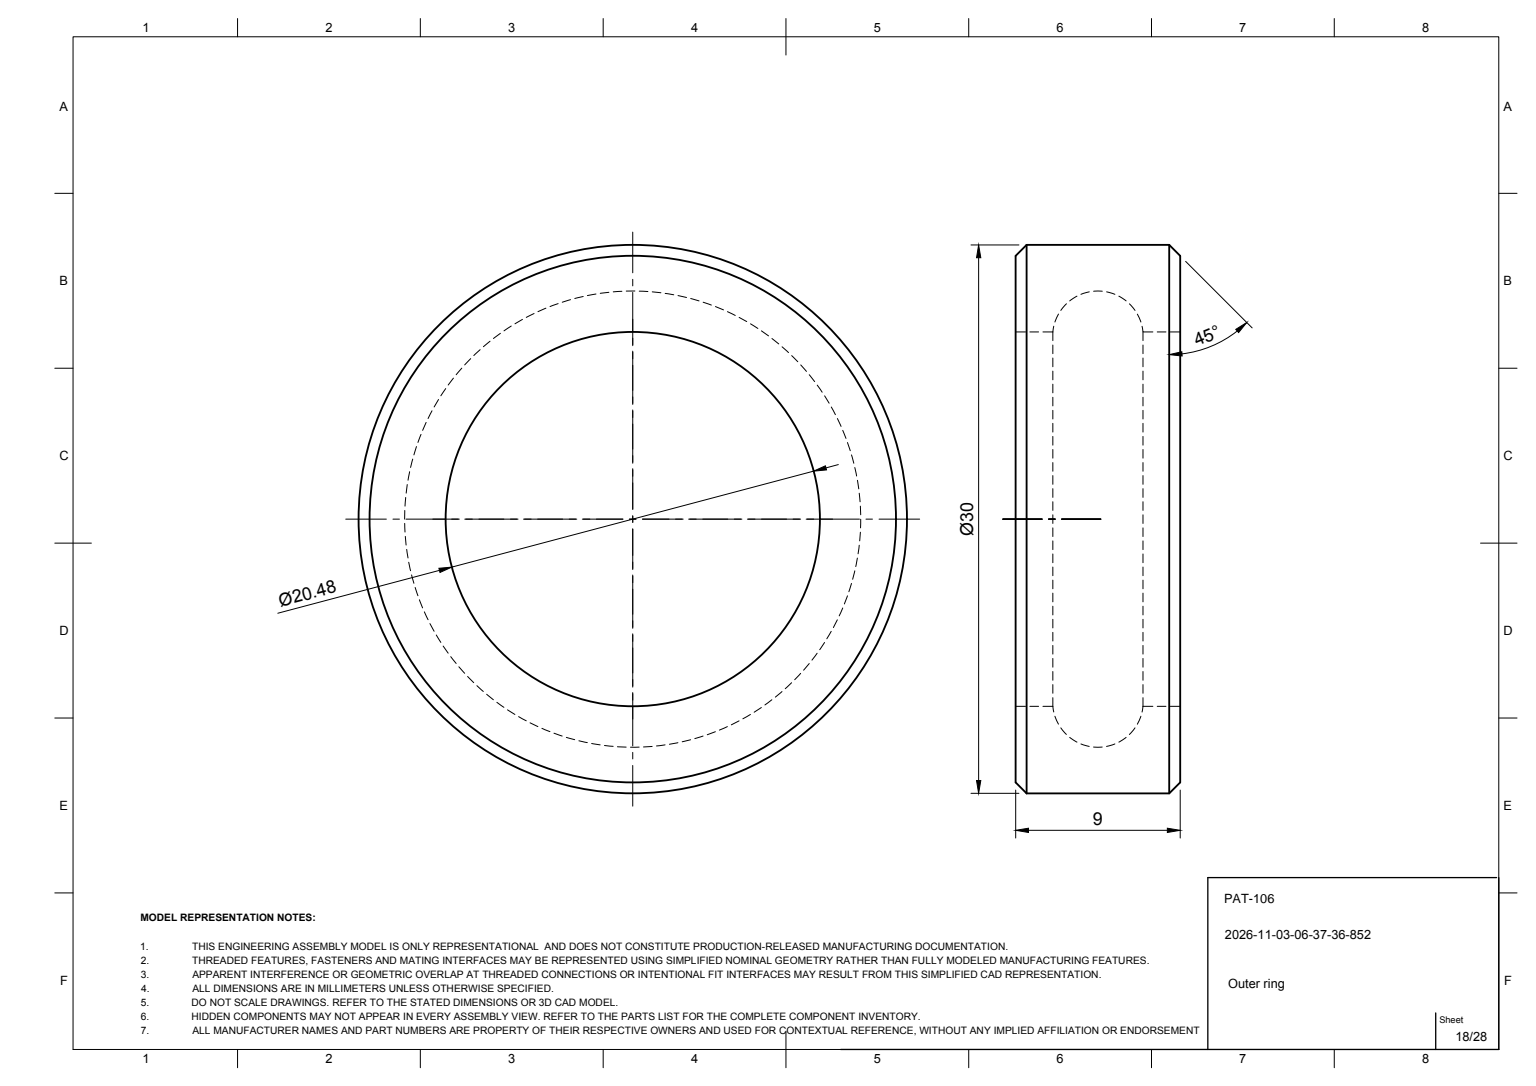
ISO-10303-21;
HEADER;
/* Generated by software containing ST-Developer
 * from STEP Tools, Inc. (www.steptools.com) 
 */

FILE_DESCRIPTION(
/* description */ ('Torsion-spring ratchet demonstrator'),
/* implementation_level */ '2;1');

FILE_NAME(
/* name */ 'Outer ring.step',
/* time_stamp */ '2026-10-29T17:29:17-07:00',
/* author */ (''),
/* organization */ (''),
/* preprocessor_version */ 'ST-DEVELOPER v20.2',
/* originating_system */ 'Autodesk Translation Framework v15.17.0.0',
/* authorisation */ '');

FILE_SCHEMA (('AUTOMOTIVE_DESIGN { 1 0 10303 214 3 1 1 }'));
ENDSEC;

DATA;
#10=MECHANICAL_DESIGN_GEOMETRIC_PRESENTATION_REPRESENTATION('',(#293),#11258);
#188=CONICAL_SURFACE('',#5713,1.47,0.785398163397449);
#189=CONICAL_SURFACE('',#5717,1.47,0.785398163397449);
#200=TOROIDAL_SURFACE('',#5702,1.,0.247676);
#245=SHAPE_REPRESENTATION_RELATIONSHIP('SRR','None',#11372,#269);
#269=ADVANCED_BREP_SHAPE_REPRESENTATION('',(#325),#11242);
#293=STYLED_ITEM('',(#11584),#325);
#325=MANIFOLD_SOLID_BREP('Body1',#5164);
#411=FACE_BOUND('',#1109,.T.);
#412=FACE_BOUND('',#1114,.T.);
#491=PLANE('',#5710);
#492=PLANE('',#5719);
#735=FACE_OUTER_BOUND('',#1106,.T.);
#736=FACE_OUTER_BOUND('',#1107,.T.);
#737=FACE_OUTER_BOUND('',#1108,.T.);
#738=FACE_OUTER_BOUND('',#1110,.T.);
#739=FACE_OUTER_BOUND('',#1111,.T.);
#740=FACE_OUTER_BOUND('',#1112,.T.);
#741=FACE_OUTER_BOUND('',#1113,.T.);
#742=FACE_OUTER_BOUND('',#1115,.T.);
#1106=EDGE_LOOP('',(#3894,#3895,#3896,#3897,#3898,#3899));
#1107=EDGE_LOOP('',(#3900,#3901,#3902,#3903,#3904));
#1108=EDGE_LOOP('',(#3905));
#1109=EDGE_LOOP('',(#3906));
#1110=EDGE_LOOP('',(#3907,#3908,#3909,#3910));
#1111=EDGE_LOOP('',(#3911,#3912,#3913,#3914));
#1112=EDGE_LOOP('',(#3915,#3916,#3917,#3918));
#1113=EDGE_LOOP('',(#3919));
#1114=EDGE_LOOP('',(#3920));
#1115=EDGE_LOOP('',(#3921,#3922,#3923,#3924,#3925));
#1424=LINE('',#8258,#1807);
#1425=LINE('',#8267,#1808);
#1426=LINE('',#8271,#1809);
#1427=LINE('',#8275,#1810);
#1428=LINE('',#8278,#1811);
#1807=VECTOR('',#6679,1.023815);
#1808=VECTOR('',#6690,1.47);
#1809=VECTOR('',#6695,1.5);
#1810=VECTOR('',#6700,1.47);
#1811=VECTOR('',#6705,1.023815);
#2214=CIRCLE('',#5703,1.023815);
#2215=CIRCLE('',#5704,1.023815);
#2216=CIRCLE('',#5705,0.247676);
#2217=CIRCLE('',#5706,1.023815);
#2218=CIRCLE('',#5707,1.023815);
#2219=CIRCLE('',#5709,1.023815);
#2220=CIRCLE('',#5711,1.44);
#2221=CIRCLE('',#5712,1.023815);
#2222=CIRCLE('',#5714,1.5);
#2223=CIRCLE('',#5716,1.5);
#2224=CIRCLE('',#5718,1.44);
#2485=VERTEX_POINT('',#8246);
#2486=VERTEX_POINT('',#8247);
#2487=VERTEX_POINT('',#8250);
#2488=VERTEX_POINT('',#8252);
#2489=VERTEX_POINT('',#8256);
#2490=VERTEX_POINT('',#8260);
#2491=VERTEX_POINT('',#8262);
#2492=VERTEX_POINT('',#8265);
#2493=VERTEX_POINT('',#8269);
#2494=VERTEX_POINT('',#8273);
#3007=EDGE_CURVE('',#2485,#2486,#2214,.T.);
#3008=EDGE_CURVE('',#2486,#2485,#2215,.T.);
#3009=EDGE_CURVE('',#2486,#2487,#2216,.T.);
#3010=EDGE_CURVE('',#2488,#2487,#2217,.T.);
#3011=EDGE_CURVE('',#2487,#2488,#2218,.T.);
#3012=EDGE_CURVE('',#2489,#2489,#2219,.T.);
#3013=EDGE_CURVE('',#2489,#2488,#1424,.T.);
#3014=EDGE_CURVE('',#2490,#2490,#2220,.T.);
#3015=EDGE_CURVE('',#2491,#2491,#2221,.T.);
#3016=EDGE_CURVE('',#2492,#2492,#2222,.T.);
#3017=EDGE_CURVE('',#2492,#2490,#1425,.T.);
#3018=EDGE_CURVE('',#2493,#2493,#2223,.T.);
#3019=EDGE_CURVE('',#2493,#2492,#1426,.T.);
#3020=EDGE_CURVE('',#2494,#2494,#2224,.T.);
#3021=EDGE_CURVE('',#2494,#2493,#1427,.T.);
#3022=EDGE_CURVE('',#2485,#2491,#1428,.T.);
#3894=ORIENTED_EDGE('',*,*,#3007,.F.);
#3895=ORIENTED_EDGE('',*,*,#3008,.F.);
#3896=ORIENTED_EDGE('',*,*,#3009,.T.);
#3897=ORIENTED_EDGE('',*,*,#3010,.F.);
#3898=ORIENTED_EDGE('',*,*,#3011,.F.);
#3899=ORIENTED_EDGE('',*,*,#3009,.F.);
#3900=ORIENTED_EDGE('',*,*,#3012,.T.);
#3901=ORIENTED_EDGE('',*,*,#3013,.T.);
#3902=ORIENTED_EDGE('',*,*,#3010,.T.);
#3903=ORIENTED_EDGE('',*,*,#3011,.T.);
#3904=ORIENTED_EDGE('',*,*,#3013,.F.);
#3905=ORIENTED_EDGE('',*,*,#3014,.F.);
#3906=ORIENTED_EDGE('',*,*,#3015,.T.);
#3907=ORIENTED_EDGE('',*,*,#3016,.F.);
#3908=ORIENTED_EDGE('',*,*,#3017,.T.);
#3909=ORIENTED_EDGE('',*,*,#3014,.T.);
#3910=ORIENTED_EDGE('',*,*,#3017,.F.);
#3911=ORIENTED_EDGE('',*,*,#3018,.F.);
#3912=ORIENTED_EDGE('',*,*,#3019,.T.);
#3913=ORIENTED_EDGE('',*,*,#3016,.T.);
#3914=ORIENTED_EDGE('',*,*,#3019,.F.);
#3915=ORIENTED_EDGE('',*,*,#3020,.F.);
#3916=ORIENTED_EDGE('',*,*,#3021,.T.);
#3917=ORIENTED_EDGE('',*,*,#3018,.T.);
#3918=ORIENTED_EDGE('',*,*,#3021,.F.);
#3919=ORIENTED_EDGE('',*,*,#3020,.T.);
#3920=ORIENTED_EDGE('',*,*,#3012,.F.);
#3921=ORIENTED_EDGE('',*,*,#3007,.T.);
#3922=ORIENTED_EDGE('',*,*,#3008,.T.);
#3923=ORIENTED_EDGE('',*,*,#3022,.T.);
#3924=ORIENTED_EDGE('',*,*,#3015,.F.);
#3925=ORIENTED_EDGE('',*,*,#3022,.F.);
#4819=CYLINDRICAL_SURFACE('',#5708,1.023815);
#4820=CYLINDRICAL_SURFACE('',#5715,1.5);
#4821=CYLINDRICAL_SURFACE('',#5720,1.023815);
#4961=ADVANCED_FACE('',(#735),#200,.F.);
#4962=ADVANCED_FACE('',(#736),#4819,.F.);
#4963=ADVANCED_FACE('',(#737,#411),#491,.T.);
#4964=ADVANCED_FACE('',(#738),#188,.T.);
#4965=ADVANCED_FACE('',(#739),#4820,.T.);
#4966=ADVANCED_FACE('',(#740),#189,.T.);
#4967=ADVANCED_FACE('',(#741,#412),#492,.T.);
#4968=ADVANCED_FACE('',(#742),#4821,.F.);
#5164=CLOSED_SHELL('',(#4961,#4962,#4963,#4964,#4965,#4966,#4967,#4968));
#5701=AXIS2_PLACEMENT_3D('',#8244,#6661,#6662);
#5702=AXIS2_PLACEMENT_3D('',#8245,#6663,#6664);
#5703=AXIS2_PLACEMENT_3D('',#8248,#6665,#6666);
#5704=AXIS2_PLACEMENT_3D('',#8249,#6667,#6668);
#5705=AXIS2_PLACEMENT_3D('',#8251,#6669,#6670);
#5706=AXIS2_PLACEMENT_3D('',#8253,#6671,#6672);
#5707=AXIS2_PLACEMENT_3D('',#8254,#6673,#6674);
#5708=AXIS2_PLACEMENT_3D('',#8255,#6675,#6676);
#5709=AXIS2_PLACEMENT_3D('',#8257,#6677,#6678);
#5710=AXIS2_PLACEMENT_3D('',#8259,#6680,#6681);
#5711=AXIS2_PLACEMENT_3D('',#8261,#6682,#6683);
#5712=AXIS2_PLACEMENT_3D('',#8263,#6684,#6685);
#5713=AXIS2_PLACEMENT_3D('',#8264,#6686,#6687);
#5714=AXIS2_PLACEMENT_3D('',#8266,#6688,#6689);
#5715=AXIS2_PLACEMENT_3D('',#8268,#6691,#6692);
#5716=AXIS2_PLACEMENT_3D('',#8270,#6693,#6694);
#5717=AXIS2_PLACEMENT_3D('',#8272,#6696,#6697);
#5718=AXIS2_PLACEMENT_3D('',#8274,#6698,#6699);
#5719=AXIS2_PLACEMENT_3D('',#8276,#6701,#6702);
#5720=AXIS2_PLACEMENT_3D('',#8277,#6703,#6704);
#6661=DIRECTION('axis',(0.,0.,1.));
#6662=DIRECTION('refdir',(1.,0.,0.));
#6663=DIRECTION('center_axis',(0.,-1.,0.));
#6664=DIRECTION('ref_axis',(0.,0.,-1.));
#6665=DIRECTION('center_axis',(0.,-1.,0.));
#6666=DIRECTION('ref_axis',(1.,0.,0.));
#6667=DIRECTION('center_axis',(0.,-1.,0.));
#6668=DIRECTION('ref_axis',(1.,0.,0.));
#6669=DIRECTION('center_axis',(1.,0.,1.22464679914735E-16));
#6670=DIRECTION('ref_axis',(-1.22464679914735E-16,0.,1.));
#6671=DIRECTION('center_axis',(0.,1.,0.));
#6672=DIRECTION('ref_axis',(1.,0.,0.));
#6673=DIRECTION('center_axis',(0.,1.,0.));
#6674=DIRECTION('ref_axis',(1.,0.,0.));
#6675=DIRECTION('center_axis',(0.,-1.,0.));
#6676=DIRECTION('ref_axis',(1.,0.,0.));
#6677=DIRECTION('center_axis',(0.,-1.,0.));
#6678=DIRECTION('ref_axis',(1.,0.,0.));
#6679=DIRECTION('',(0.,1.,0.));
#6680=DIRECTION('center_axis',(0.,1.,0.));
#6681=DIRECTION('ref_axis',(0.,0.,1.));
#6682=DIRECTION('center_axis',(0.,-1.,0.));
#6683=DIRECTION('ref_axis',(1.,0.,0.));
#6684=DIRECTION('center_axis',(0.,-1.,0.));
#6685=DIRECTION('ref_axis',(1.,0.,0.));
#6686=DIRECTION('center_axis',(0.,-1.,0.));
#6687=DIRECTION('ref_axis',(1.,0.,0.));
#6688=DIRECTION('center_axis',(0.,-1.,0.));
#6689=DIRECTION('ref_axis',(1.,0.,0.));
#6690=DIRECTION('',(0.707106781186548,0.707106781186547,8.65956056235494E-17));
#6691=DIRECTION('center_axis',(0.,-1.,0.));
#6692=DIRECTION('ref_axis',(1.,0.,0.));
#6693=DIRECTION('center_axis',(0.,-1.,0.));
#6694=DIRECTION('ref_axis',(1.,0.,0.));
#6695=DIRECTION('',(0.,1.,0.));
#6696=DIRECTION('center_axis',(0.,1.,0.));
#6697=DIRECTION('ref_axis',(1.,0.,0.));
#6698=DIRECTION('center_axis',(0.,-1.,0.));
#6699=DIRECTION('ref_axis',(1.,0.,0.));
#6700=DIRECTION('',(-0.707106781186548,0.707106781186547,-8.65956056235494E-17));
#6701=DIRECTION('center_axis',(0.,-1.,0.));
#6702=DIRECTION('ref_axis',(0.,0.,-1.));
#6703=DIRECTION('center_axis',(0.,-1.,0.));
#6704=DIRECTION('ref_axis',(1.,0.,0.));
#6705=DIRECTION('',(0.,1.,0.));
#8244=CARTESIAN_POINT('',(0.,0.,0.));
#8245=CARTESIAN_POINT('Origin',(0.,0.,0.));
#8246=CARTESIAN_POINT('',(-1.023815,0.246528389340863,-1.25381176266905E-16));
#8247=CARTESIAN_POINT('',(-1.25381176266905E-16,0.246528389340863,1.023815));
#8248=CARTESIAN_POINT('Origin',(0.,0.246528389340863,0.));
#8249=CARTESIAN_POINT('Origin',(0.,0.246528389340863,0.));
#8250=CARTESIAN_POINT('',(-1.25381176266905E-16,-0.246528389340863,1.023815));
#8251=CARTESIAN_POINT('Origin',(-1.22464679914735E-16,0.,1.));
#8252=CARTESIAN_POINT('',(-1.023815,-0.246528389340863,1.25381176266905E-16));
#8253=CARTESIAN_POINT('Origin',(0.,-0.246528389340863,0.));
#8254=CARTESIAN_POINT('Origin',(0.,-0.246528389340863,0.));
#8255=CARTESIAN_POINT('Origin',(0.,0.,0.));
#8256=CARTESIAN_POINT('',(-1.023815,-0.45,-1.25381176266905E-16));
#8257=CARTESIAN_POINT('Origin',(0.,-0.45,0.));
#8258=CARTESIAN_POINT('',(-1.023815,0.,-1.25381176266905E-16));
#8259=CARTESIAN_POINT('Origin',(1.44,0.45,0.));
#8260=CARTESIAN_POINT('',(-1.44,0.45,-1.76349139077219E-16));
#8261=CARTESIAN_POINT('Origin',(0.,0.45,0.));
#8262=CARTESIAN_POINT('',(-1.023815,0.45,-1.25381176266905E-16));
#8263=CARTESIAN_POINT('Origin',(0.,0.45,0.));
#8264=CARTESIAN_POINT('Origin',(0.,0.42,0.));
#8265=CARTESIAN_POINT('',(-1.5,0.39,-1.83697019872103E-16));
#8266=CARTESIAN_POINT('Origin',(0.,0.39,0.));
#8267=CARTESIAN_POINT('',(-1.47,0.42,-1.80023079474661E-16));
#8268=CARTESIAN_POINT('Origin',(0.,0.,0.));
#8269=CARTESIAN_POINT('',(-1.5,-0.39,-1.83697019872103E-16));
#8270=CARTESIAN_POINT('Origin',(0.,-0.39,0.));
#8271=CARTESIAN_POINT('',(-1.5,0.,-1.83697019872103E-16));
#8272=CARTESIAN_POINT('Origin',(0.,-0.42,0.));
#8273=CARTESIAN_POINT('',(-1.44,-0.45,-1.76349139077219E-16));
#8274=CARTESIAN_POINT('Origin',(0.,-0.45,0.));
#8275=CARTESIAN_POINT('',(-1.47,-0.42,-1.80023079474661E-16));
#8276=CARTESIAN_POINT('Origin',(1.023815,-0.45,0.));
#8277=CARTESIAN_POINT('Origin',(0.,0.,0.));
#8278=CARTESIAN_POINT('',(-1.023815,0.,-1.25381176266905E-16));
#11212=UNCERTAINTY_MEASURE_WITH_UNIT(LENGTH_MEASURE(0.001),#11259,
'DISTANCE_ACCURACY_VALUE',
'Maximum model space distance between geometric entities at asserted c
onnectivities');
#11228=UNCERTAINTY_MEASURE_WITH_UNIT(LENGTH_MEASURE(0.001),#11259,
'DISTANCE_ACCURACY_VALUE',
'Maximum model space distance between geometric entities at asserted c
onnectivities');
#11242=(
GEOMETRIC_REPRESENTATION_CONTEXT(3)
GLOBAL_UNCERTAINTY_ASSIGNED_CONTEXT((#11212))
GLOBAL_UNIT_ASSIGNED_CONTEXT((#11259,#11261,#11262))
REPRESENTATION_CONTEXT('','3D')
);
#11258=(
GEOMETRIC_REPRESENTATION_CONTEXT(3)
GLOBAL_UNCERTAINTY_ASSIGNED_CONTEXT((#11228))
GLOBAL_UNIT_ASSIGNED_CONTEXT((#11259,#11261,#11262))
REPRESENTATION_CONTEXT('','3D')
);
#11259=(
LENGTH_UNIT()
NAMED_UNIT(*)
SI_UNIT(.CENTI.,.METRE.)
);
#11261=(
NAMED_UNIT(*)
PLANE_ANGLE_UNIT()
SI_UNIT($,.RADIAN.)
);
#11262=(
NAMED_UNIT(*)
SI_UNIT($,.STERADIAN.)
SOLID_ANGLE_UNIT()
);
#11276=SHAPE_DEFINITION_REPRESENTATION(#11305,#11372);
#11305=PRODUCT_DEFINITION_SHAPE('',$,#11402);
#11372=SHAPE_REPRESENTATION('',(#5701),#11242);
#11388=PRODUCT_DEFINITION_CONTEXT('part definition',#11477,'design');
#11402=PRODUCT_DEFINITION('Outer ring','Outer ring',#11431,#11388);
#11431=PRODUCT_DEFINITION_FORMATION('',$,#11492);
#11477=APPLICATION_CONTEXT(
'Core Data for Automotive Mechanical Design Process');
#11478=PRODUCT_CONTEXT('part definition',#11477,'mechanical');
#11492=PRODUCT('Outer ring','Outer ring','Outer ring',(#11478));
#11578=COLOUR_RGB('Grey',0.48,0.52,0.57);
#11579=FILL_AREA_STYLE_COLOUR('',#11578);
#11580=FILL_AREA_STYLE('',(#11579));
#11581=SURFACE_STYLE_FILL_AREA(#11580);
#11582=SURFACE_SIDE_STYLE('',(#11581));
#11583=SURFACE_STYLE_USAGE(.BOTH.,#11582);
#11584=PRESENTATION_STYLE_ASSIGNMENT((#11583));
ENDSEC;
END-ISO-10303-21;
